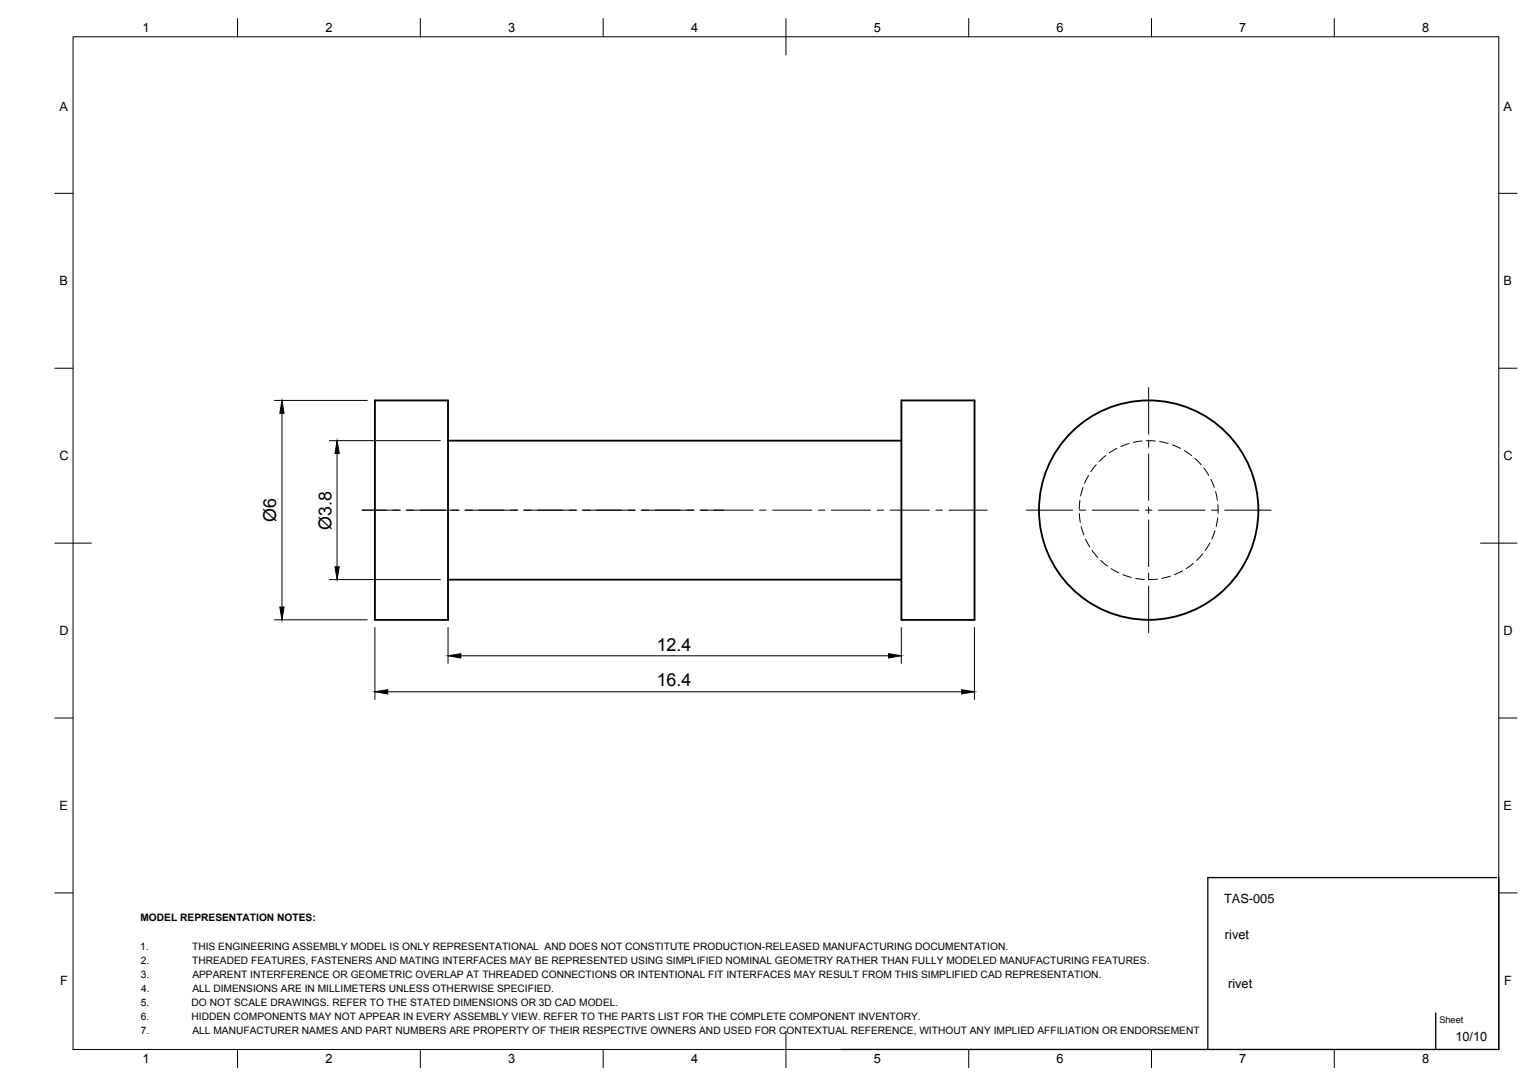
ISO-10303-21;
HEADER;
/* Generated by software containing ST-Developer
 * from STEP Tools, Inc. (www.steptools.com) 
 */

FILE_DESCRIPTION(
/* description */ ('STEP AP214'),
/* implementation_level */ '2;1');

FILE_NAME(
/* name */ 'rivet.step',
/* time_stamp */ '2026-11-04T19:54:22-08:00',
/* author */ (''),
/* organization */ (''),
/* preprocessor_version */ 'ST-DEVELOPER v20.2',
/* originating_system */ 'Autodesk Translation Framework v15.17.0.0',
/* authorisation */ '');

FILE_SCHEMA (('AUTOMOTIVE_DESIGN { 1 0 10303 214 3 1 1 }'));
ENDSEC;

DATA;
#10=MECHANICAL_DESIGN_GEOMETRIC_PRESENTATION_REPRESENTATION('',(#247),#14084);
#229=SHAPE_REPRESENTATION_RELATIONSHIP('SRR','None',#14128,#238);
#238=ADVANCED_BREP_SHAPE_REPRESENTATION('',(#256),#14083);
#247=STYLED_ITEM('',(#14178),#256);
#256=MANIFOLD_SOLID_BREP('Body1',#3473);
#283=FACE_BOUND('',#769,.T.);
#284=FACE_BOUND('',#772,.T.);
#361=PLANE('',#3850);
#362=PLANE('',#3851);
#363=PLANE('',#3852);
#364=PLANE('',#3853);
#548=FACE_OUTER_BOUND('',#764,.T.);
#549=FACE_OUTER_BOUND('',#765,.T.);
#550=FACE_OUTER_BOUND('',#766,.T.);
#551=FACE_OUTER_BOUND('',#767,.T.);
#552=FACE_OUTER_BOUND('',#768,.T.);
#553=FACE_OUTER_BOUND('',#770,.T.);
#554=FACE_OUTER_BOUND('',#771,.T.);
#764=EDGE_LOOP('',(#3169,#3170,#3171,#3172));
#765=EDGE_LOOP('',(#3173,#3174,#3175,#3176));
#766=EDGE_LOOP('',(#3177,#3178,#3179,#3180));
#767=EDGE_LOOP('',(#3181));
#768=EDGE_LOOP('',(#3182));
#769=EDGE_LOOP('',(#3183));
#770=EDGE_LOOP('',(#3184));
#771=EDGE_LOOP('',(#3185));
#772=EDGE_LOOP('',(#3186));
#1027=LINE('',#14035,#1284);
#1028=LINE('',#14041,#1285);
#1029=LINE('',#14047,#1286);
#1284=VECTOR('',#4656,3.);
#1285=VECTOR('',#4663,3.);
#1286=VECTOR('',#4670,1.9);
#1371=CIRCLE('',#3842,3.);
#1372=CIRCLE('',#3843,3.);
#1373=CIRCLE('',#3845,3.);
#1374=CIRCLE('',#3846,3.);
#1375=CIRCLE('',#3848,1.9);
#1376=CIRCLE('',#3849,1.9);
#1696=VERTEX_POINT('',#14032);
#1697=VERTEX_POINT('',#14034);
#1698=VERTEX_POINT('',#14038);
#1699=VERTEX_POINT('',#14040);
#1700=VERTEX_POINT('',#14044);
#1701=VERTEX_POINT('',#14046);
#2188=EDGE_CURVE('',#1696,#1696,#1371,.T.);
#2189=EDGE_CURVE('',#1696,#1697,#1027,.T.);
#2190=EDGE_CURVE('',#1697,#1697,#1372,.T.);
#2191=EDGE_CURVE('',#1698,#1698,#1373,.T.);
#2192=EDGE_CURVE('',#1698,#1699,#1028,.T.);
#2193=EDGE_CURVE('',#1699,#1699,#1374,.T.);
#2194=EDGE_CURVE('',#1700,#1700,#1375,.T.);
#2195=EDGE_CURVE('',#1700,#1701,#1029,.T.);
#2196=EDGE_CURVE('',#1701,#1701,#1376,.T.);
#3169=ORIENTED_EDGE('',*,*,#2188,.T.);
#3170=ORIENTED_EDGE('',*,*,#2189,.T.);
#3171=ORIENTED_EDGE('',*,*,#2190,.F.);
#3172=ORIENTED_EDGE('',*,*,#2189,.F.);
#3173=ORIENTED_EDGE('',*,*,#2191,.T.);
#3174=ORIENTED_EDGE('',*,*,#2192,.T.);
#3175=ORIENTED_EDGE('',*,*,#2193,.F.);
#3176=ORIENTED_EDGE('',*,*,#2192,.F.);
#3177=ORIENTED_EDGE('',*,*,#2194,.F.);
#3178=ORIENTED_EDGE('',*,*,#2195,.T.);
#3179=ORIENTED_EDGE('',*,*,#2196,.F.);
#3180=ORIENTED_EDGE('',*,*,#2195,.F.);
#3181=ORIENTED_EDGE('',*,*,#2193,.T.);
#3182=ORIENTED_EDGE('',*,*,#2191,.F.);
#3183=ORIENTED_EDGE('',*,*,#2194,.T.);
#3184=ORIENTED_EDGE('',*,*,#2190,.T.);
#3185=ORIENTED_EDGE('',*,*,#2188,.F.);
#3186=ORIENTED_EDGE('',*,*,#2196,.T.);
#3272=CYLINDRICAL_SURFACE('',#3841,3.);
#3273=CYLINDRICAL_SURFACE('',#3844,3.);
#3274=CYLINDRICAL_SURFACE('',#3847,1.9);
#3458=ADVANCED_FACE('',(#548),#3272,.T.);
#3459=ADVANCED_FACE('',(#549),#3273,.T.);
#3460=ADVANCED_FACE('',(#550),#3274,.T.);
#3461=ADVANCED_FACE('',(#551),#361,.T.);
#3462=ADVANCED_FACE('',(#552,#283),#362,.F.);
#3463=ADVANCED_FACE('',(#553),#363,.T.);
#3464=ADVANCED_FACE('',(#554,#284),#364,.F.);
#3473=CLOSED_SHELL('',(#3458,#3459,#3460,#3461,#3462,#3463,#3464));
#3840=AXIS2_PLACEMENT_3D('',#14030,#4650,#4651);
#3841=AXIS2_PLACEMENT_3D('',#14031,#4652,#4653);
#3842=AXIS2_PLACEMENT_3D('',#14033,#4654,#4655);
#3843=AXIS2_PLACEMENT_3D('',#14036,#4657,#4658);
#3844=AXIS2_PLACEMENT_3D('',#14037,#4659,#4660);
#3845=AXIS2_PLACEMENT_3D('',#14039,#4661,#4662);
#3846=AXIS2_PLACEMENT_3D('',#14042,#4664,#4665);
#3847=AXIS2_PLACEMENT_3D('',#14043,#4666,#4667);
#3848=AXIS2_PLACEMENT_3D('',#14045,#4668,#4669);
#3849=AXIS2_PLACEMENT_3D('',#14048,#4671,#4672);
#3850=AXIS2_PLACEMENT_3D('',#14049,#4673,#4674);
#3851=AXIS2_PLACEMENT_3D('',#14050,#4675,#4676);
#3852=AXIS2_PLACEMENT_3D('',#14051,#4677,#4678);
#3853=AXIS2_PLACEMENT_3D('',#14052,#4679,#4680);
#4650=DIRECTION('axis',(0.,0.,1.));
#4651=DIRECTION('refdir',(1.,0.,0.));
#4652=DIRECTION('center_axis',(0.,0.,1.));
#4653=DIRECTION('ref_axis',(1.,0.,0.));
#4654=DIRECTION('center_axis',(0.,0.,-1.));
#4655=DIRECTION('ref_axis',(-1.,0.,0.));
#4656=DIRECTION('',(0.,0.,-1.));
#4657=DIRECTION('center_axis',(0.,0.,-1.));
#4658=DIRECTION('ref_axis',(-1.,0.,0.));
#4659=DIRECTION('center_axis',(0.,0.,-1.));
#4660=DIRECTION('ref_axis',(-1.,0.,0.));
#4661=DIRECTION('center_axis',(0.,0.,1.));
#4662=DIRECTION('ref_axis',(1.,0.,0.));
#4663=DIRECTION('',(0.,0.,1.));
#4664=DIRECTION('center_axis',(0.,0.,1.));
#4665=DIRECTION('ref_axis',(1.,0.,0.));
#4666=DIRECTION('center_axis',(0.,0.,1.));
#4667=DIRECTION('ref_axis',(1.,0.,0.));
#4668=DIRECTION('center_axis',(0.,0.,1.));
#4669=DIRECTION('ref_axis',(1.,0.,0.));
#4670=DIRECTION('',(0.,0.,-1.));
#4671=DIRECTION('center_axis',(0.,0.,-1.));
#4672=DIRECTION('ref_axis',(1.,0.,0.));
#4673=DIRECTION('center_axis',(0.,0.,1.));
#4674=DIRECTION('ref_axis',(1.,0.,0.));
#4675=DIRECTION('center_axis',(0.,0.,1.));
#4676=DIRECTION('ref_axis',(1.,0.,0.));
#4677=DIRECTION('center_axis',(0.,0.,-1.));
#4678=DIRECTION('ref_axis',(-1.,0.,0.));
#4679=DIRECTION('center_axis',(0.,0.,-1.));
#4680=DIRECTION('ref_axis',(-1.,0.,0.));
#14030=CARTESIAN_POINT('',(0.,0.,0.));
#14031=CARTESIAN_POINT('Origin',(32.,329.539392014169,-8.2));
#14032=CARTESIAN_POINT('',(29.,329.539392014169,-6.2));
#14033=CARTESIAN_POINT('Origin',(32.,329.539392014169,-6.2));
#14034=CARTESIAN_POINT('',(29.,329.539392014169,-8.2));
#14035=CARTESIAN_POINT('',(29.,329.539392014169,-8.2));
#14036=CARTESIAN_POINT('Origin',(32.,329.539392014169,-8.2));
#14037=CARTESIAN_POINT('Origin',(32.,329.539392014169,8.2));
#14038=CARTESIAN_POINT('',(35.,329.539392014169,6.2));
#14039=CARTESIAN_POINT('Origin',(32.,329.539392014169,6.2));
#14040=CARTESIAN_POINT('',(35.,329.539392014169,8.2));
#14041=CARTESIAN_POINT('',(35.,329.539392014169,8.2));
#14042=CARTESIAN_POINT('Origin',(32.,329.539392014169,8.2));
#14043=CARTESIAN_POINT('Origin',(32.,329.539392014169,-11.5740115370178));
#14044=CARTESIAN_POINT('',(30.1,329.539392014169,6.2));
#14045=CARTESIAN_POINT('Origin',(32.,329.539392014169,6.2));
#14046=CARTESIAN_POINT('',(30.1,329.539392014169,-6.2));
#14047=CARTESIAN_POINT('',(30.1,329.539392014169,-11.5740115370178));
#14048=CARTESIAN_POINT('Origin',(32.,329.539392014169,-6.2));
#14049=CARTESIAN_POINT('Origin',(32.,329.539392014169,8.2));
#14050=CARTESIAN_POINT('Origin',(32.,329.539392014169,6.2));
#14051=CARTESIAN_POINT('Origin',(32.,329.539392014169,-8.2));
#14052=CARTESIAN_POINT('Origin',(32.,329.539392014169,-6.2));
#14072=UNCERTAINTY_MEASURE_WITH_UNIT(LENGTH_MEASURE(0.01),#14085,
'DISTANCE_ACCURACY_VALUE',
'Maximum model space distance between geometric entities at asserted c
onnectivities');
#14073=UNCERTAINTY_MEASURE_WITH_UNIT(LENGTH_MEASURE(0.01),#14085,
'DISTANCE_ACCURACY_VALUE',
'Maximum model space distance between geometric entities at asserted c
onnectivities');
#14083=(
GEOMETRIC_REPRESENTATION_CONTEXT(3)
GLOBAL_UNCERTAINTY_ASSIGNED_CONTEXT((#14072))
GLOBAL_UNIT_ASSIGNED_CONTEXT((#14085,#14087,#14088))
REPRESENTATION_CONTEXT('','3D')
);
#14084=(
GEOMETRIC_REPRESENTATION_CONTEXT(3)
GLOBAL_UNCERTAINTY_ASSIGNED_CONTEXT((#14073))
GLOBAL_UNIT_ASSIGNED_CONTEXT((#14085,#14087,#14088))
REPRESENTATION_CONTEXT('','3D')
);
#14085=(
LENGTH_UNIT()
NAMED_UNIT(*)
SI_UNIT(.MILLI.,.METRE.)
);
#14087=(
NAMED_UNIT(*)
PLANE_ANGLE_UNIT()
SI_UNIT($,.RADIAN.)
);
#14088=(
NAMED_UNIT(*)
SI_UNIT($,.STERADIAN.)
SOLID_ANGLE_UNIT()
);
#14098=SHAPE_DEFINITION_REPRESENTATION(#14108,#14128);
#14108=PRODUCT_DEFINITION_SHAPE('',$,#14139);
#14128=SHAPE_REPRESENTATION('',(#3840),#14083);
#14129=PRODUCT_DEFINITION_CONTEXT('part definition',#14161,'design');
#14139=PRODUCT_DEFINITION('rivet','rivet',#14149,#14129);
#14149=PRODUCT_DEFINITION_FORMATION('',$,#14172);
#14161=APPLICATION_CONTEXT(
'Core Data for Automotive Mechanical Design Process');
#14162=PRODUCT_CONTEXT('part definition',#14161,'mechanical');
#14172=PRODUCT('rivet','rivet',$,(#14162));
#14178=PRESENTATION_STYLE_ASSIGNMENT((#14184));
#14184=SURFACE_STYLE_USAGE(.BOTH.,#14190);
#14190=SURFACE_SIDE_STYLE('',(#14196));
#14196=SURFACE_STYLE_FILL_AREA(#14202);
#14202=FILL_AREA_STYLE('Opaque(61,176,222)',(#14208));
#14208=FILL_AREA_STYLE_COLOUR('Opaque(61,176,222)',#14214);
#14214=COLOUR_RGB('Opaque(61,176,222)',0.23921568627451,0.690196078431373,
0.870588235294118);
ENDSEC;
END-ISO-10303-21;
